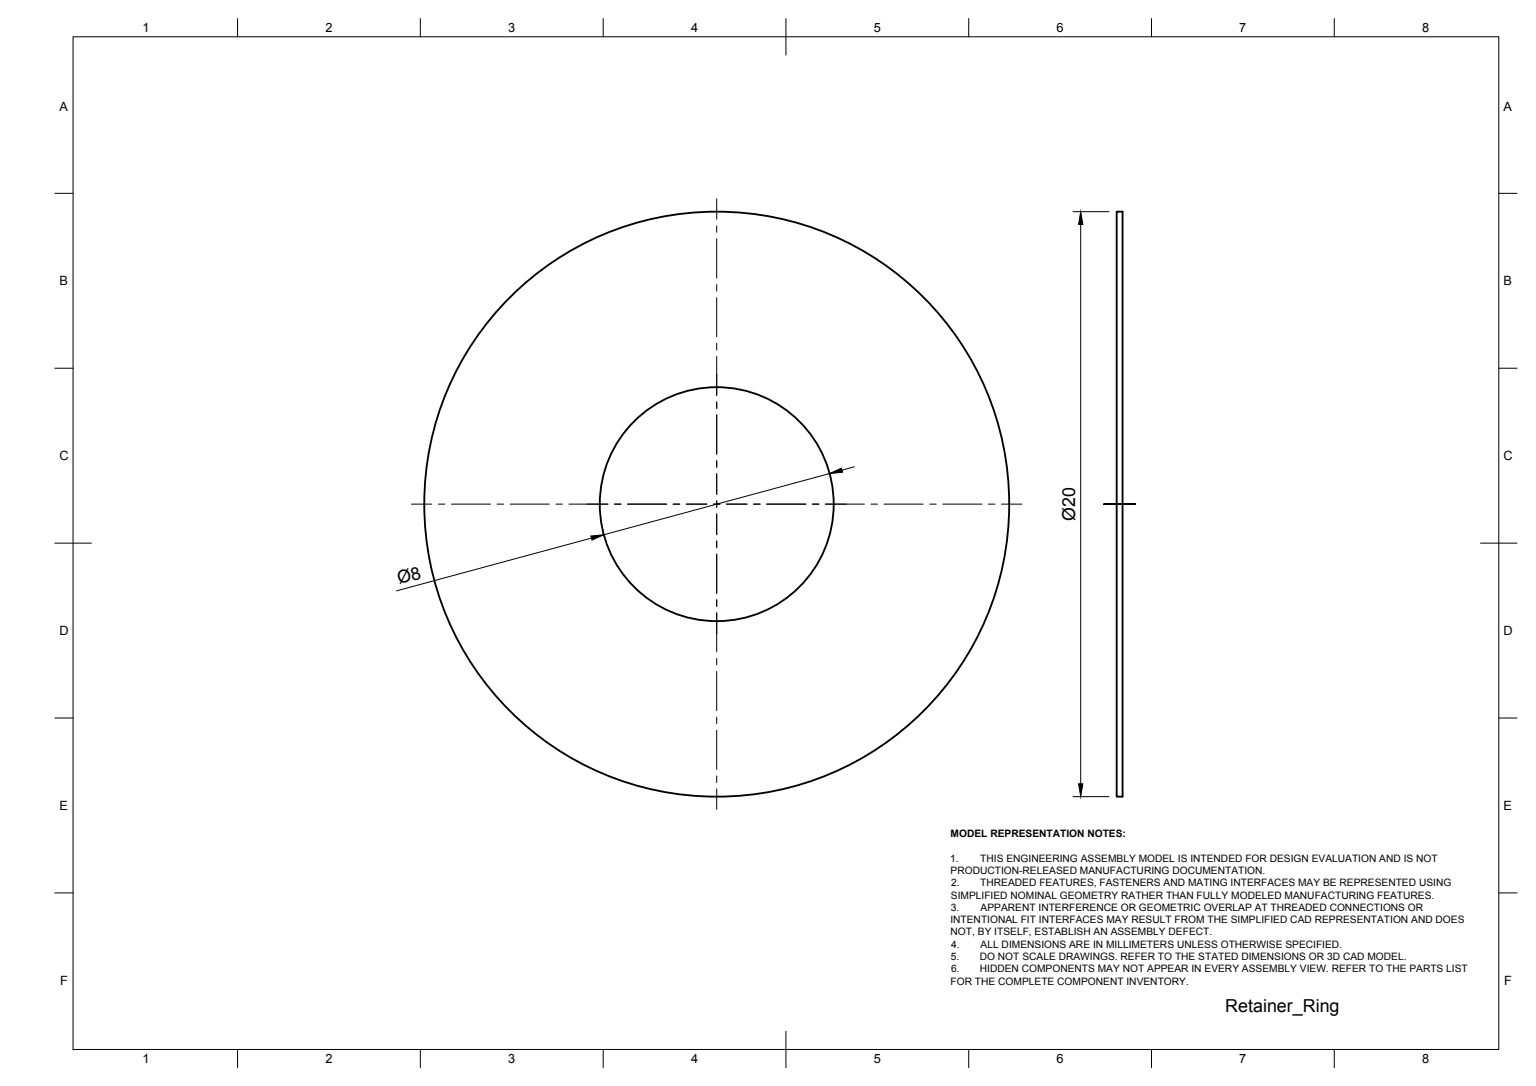
ISO-10303-21;
HEADER;
/* Generated by software containing ST-Developer
 * from STEP Tools, Inc. (www.steptools.com) 
 */

FILE_DESCRIPTION(
/* description */ (''),
/* implementation_level */ '2;1');

FILE_NAME(
/* name */ 'Retainer_Ring.step',
/* time_stamp */ '2026-10-06T12:52:28-07:00',
/* author */ (''),
/* organization */ (''),
/* preprocessor_version */ 'ST-DEVELOPER v20.2',
/* originating_system */ 'Autodesk Translation Framework v15.15.0.0',
/* authorisation */ '');

FILE_SCHEMA (('AUTOMOTIVE_DESIGN { 1 0 10303 214 3 1 1 }'));
ENDSEC;

DATA;
#10=MECHANICAL_DESIGN_GEOMETRIC_PRESENTATION_REPRESENTATION('',(#75),#34403);
#59=SHAPE_REPRESENTATION_RELATIONSHIP('SRR','None',#34437,#67);
#67=ADVANCED_BREP_SHAPE_REPRESENTATION('',(#83),#34397);
#75=STYLED_ITEM('',(#34484),#83);
#83=MANIFOLD_SOLID_BREP('Body1',#4384);
#95=FACE_BOUND('',#769,.T.);
#96=FACE_BOUND('',#771,.T.);
#129=PLANE('',#4520);
#130=PLANE('',#4521);
#178=CIRCLE('',#4515,4.);
#179=CIRCLE('',#4516,4.);
#180=CIRCLE('',#4518,10.);
#181=CIRCLE('',#4519,10.);
#529=FACE_OUTER_BOUND('',#766,.T.);
#530=FACE_OUTER_BOUND('',#767,.T.);
#531=FACE_OUTER_BOUND('',#768,.T.);
#532=FACE_OUTER_BOUND('',#770,.T.);
#766=EDGE_LOOP('',(#2745,#2746,#2747,#2748));
#767=EDGE_LOOP('',(#2749,#2750,#2751,#2752));
#768=EDGE_LOOP('',(#2753));
#769=EDGE_LOOP('',(#2754));
#770=EDGE_LOOP('',(#2755));
#771=EDGE_LOOP('',(#2756));
#1019=LINE('',#6398,#1156);
#1020=LINE('',#6404,#1157);
#1156=VECTOR('',#5082,4.);
#1157=VECTOR('',#5089,10.);
#1562=VERTEX_POINT('',#6395);
#1563=VERTEX_POINT('',#6397);
#1564=VERTEX_POINT('',#6401);
#1565=VERTEX_POINT('',#6403);
#2037=EDGE_CURVE('',#1562,#1562,#178,.T.);
#2038=EDGE_CURVE('',#1562,#1563,#1019,.T.);
#2039=EDGE_CURVE('',#1563,#1563,#179,.T.);
#2040=EDGE_CURVE('',#1564,#1564,#180,.F.);
#2041=EDGE_CURVE('',#1564,#1565,#1020,.T.);
#2042=EDGE_CURVE('',#1565,#1565,#181,.F.);
#2745=ORIENTED_EDGE('',*,*,#2037,.T.);
#2746=ORIENTED_EDGE('',*,*,#2038,.T.);
#2747=ORIENTED_EDGE('',*,*,#2039,.F.);
#2748=ORIENTED_EDGE('',*,*,#2038,.F.);
#2749=ORIENTED_EDGE('',*,*,#2040,.F.);
#2750=ORIENTED_EDGE('',*,*,#2041,.T.);
#2751=ORIENTED_EDGE('',*,*,#2042,.T.);
#2752=ORIENTED_EDGE('',*,*,#2041,.F.);
#2753=ORIENTED_EDGE('',*,*,#2040,.T.);
#2754=ORIENTED_EDGE('',*,*,#2039,.T.);
#2755=ORIENTED_EDGE('',*,*,#2042,.F.);
#2756=ORIENTED_EDGE('',*,*,#2037,.F.);
#4042=CYLINDRICAL_SURFACE('',#4514,4.);
#4043=CYLINDRICAL_SURFACE('',#4517,10.);
#4164=ADVANCED_FACE('',(#529),#4042,.F.);
#4165=ADVANCED_FACE('',(#530),#4043,.T.);
#4166=ADVANCED_FACE('',(#531,#95),#129,.T.);
#4167=ADVANCED_FACE('',(#532,#96),#130,.F.);
#4384=CLOSED_SHELL('',(#4164,#4165,#4166,#4167));
#4513=AXIS2_PLACEMENT_3D('',#6393,#5076,#5077);
#4514=AXIS2_PLACEMENT_3D('',#6394,#5078,#5079);
#4515=AXIS2_PLACEMENT_3D('',#6396,#5080,#5081);
#4516=AXIS2_PLACEMENT_3D('',#6399,#5083,#5084);
#4517=AXIS2_PLACEMENT_3D('',#6400,#5085,#5086);
#4518=AXIS2_PLACEMENT_3D('',#6402,#5087,#5088);
#4519=AXIS2_PLACEMENT_3D('',#6405,#5090,#5091);
#4520=AXIS2_PLACEMENT_3D('',#6406,#5092,#5093);
#4521=AXIS2_PLACEMENT_3D('',#6407,#5094,#5095);
#5076=DIRECTION('axis',(0.,0.,1.));
#5077=DIRECTION('refdir',(1.,0.,0.));
#5078=DIRECTION('center_axis',(0.,0.,1.));
#5079=DIRECTION('ref_axis',(-1.,0.,0.));
#5080=DIRECTION('center_axis',(0.,0.,-1.));
#5081=DIRECTION('ref_axis',(-1.,0.,0.));
#5082=DIRECTION('',(0.,0.,1.));
#5083=DIRECTION('center_axis',(0.,0.,-1.));
#5084=DIRECTION('ref_axis',(-1.,0.,0.));
#5085=DIRECTION('center_axis',(0.,0.,1.));
#5086=DIRECTION('ref_axis',(-1.,0.,0.));
#5087=DIRECTION('center_axis',(0.,0.,-1.));
#5088=DIRECTION('ref_axis',(-1.,0.,0.));
#5089=DIRECTION('',(0.,0.,-1.));
#5090=DIRECTION('center_axis',(0.,0.,-1.));
#5091=DIRECTION('ref_axis',(-1.,0.,0.));
#5092=DIRECTION('center_axis',(0.,0.,1.));
#5093=DIRECTION('ref_axis',(-1.,0.,0.));
#5094=DIRECTION('center_axis',(0.,0.,1.));
#5095=DIRECTION('ref_axis',(-1.,0.,0.));
#6393=CARTESIAN_POINT('',(0.,0.,0.));
#6394=CARTESIAN_POINT('Origin',(0.,0.,60.));
#6395=CARTESIAN_POINT('',(4.,4.89858719658941E-16,60.));
#6396=CARTESIAN_POINT('Origin',(0.,0.,60.));
#6397=CARTESIAN_POINT('',(4.,4.89858719658941E-16,60.2));
#6398=CARTESIAN_POINT('',(4.,4.89858719658941E-16,60.));
#6399=CARTESIAN_POINT('Origin',(0.,0.,60.2));
#6400=CARTESIAN_POINT('Origin',(0.,0.,60.));
#6401=CARTESIAN_POINT('',(10.,-1.22464679914735E-15,60.2));
#6402=CARTESIAN_POINT('Origin',(0.,0.,60.2));
#6403=CARTESIAN_POINT('',(10.,-1.22464679914735E-15,60.));
#6404=CARTESIAN_POINT('',(10.,1.22464679914735E-15,60.));
#6405=CARTESIAN_POINT('Origin',(0.,0.,60.));
#6406=CARTESIAN_POINT('Origin',(0.,0.,60.2));
#6407=CARTESIAN_POINT('Origin',(0.,0.,60.));
#34387=UNCERTAINTY_MEASURE_WITH_UNIT(LENGTH_MEASURE(0.01),#34404,
'DISTANCE_ACCURACY_VALUE',
'Maximum model space distance between geometric entities at asserted c
onnectivities');
#34393=UNCERTAINTY_MEASURE_WITH_UNIT(LENGTH_MEASURE(0.01),#34404,
'DISTANCE_ACCURACY_VALUE',
'Maximum model space distance between geometric entities at asserted c
onnectivities');
#34397=(
GEOMETRIC_REPRESENTATION_CONTEXT(3)
GLOBAL_UNCERTAINTY_ASSIGNED_CONTEXT((#34387))
GLOBAL_UNIT_ASSIGNED_CONTEXT((#34404,#34406,#34407))
REPRESENTATION_CONTEXT('','3D')
);
#34403=(
GEOMETRIC_REPRESENTATION_CONTEXT(3)
GLOBAL_UNCERTAINTY_ASSIGNED_CONTEXT((#34393))
GLOBAL_UNIT_ASSIGNED_CONTEXT((#34404,#34406,#34407))
REPRESENTATION_CONTEXT('','3D')
);
#34404=(
LENGTH_UNIT()
NAMED_UNIT(*)
SI_UNIT(.MILLI.,.METRE.)
);
#34406=(
NAMED_UNIT(*)
PLANE_ANGLE_UNIT()
SI_UNIT($,.RADIAN.)
);
#34407=(
NAMED_UNIT(*)
SI_UNIT($,.STERADIAN.)
SOLID_ANGLE_UNIT()
);
#34411=SHAPE_DEFINITION_REPRESENTATION(#34420,#34437);
#34420=PRODUCT_DEFINITION_SHAPE('',$,#34447);
#34437=SHAPE_REPRESENTATION('',(#4513),#34397);
#34443=PRODUCT_DEFINITION_CONTEXT('part definition',#34472,'design');
#34447=PRODUCT_DEFINITION('Retainer_Ring','Retainer_Ring',#34456,#34443);
#34456=PRODUCT_DEFINITION_FORMATION('',$,#34477);
#34472=APPLICATION_CONTEXT(
'Core Data for Automotive Mechanical Design Process');
#34473=PRODUCT_CONTEXT('part definition',#34472,'mechanical');
#34477=PRODUCT('Retainer_Ring','Retainer_Ring',$,(#34473));
#34484=PRESENTATION_STYLE_ASSIGNMENT((#34486));
#34486=SURFACE_STYLE_USAGE(.BOTH.,#34488);
#34488=SURFACE_SIDE_STYLE('',(#34490));
#34490=SURFACE_STYLE_FILL_AREA(#34492);
#34492=FILL_AREA_STYLE('Opaque(160,160,160)',(#34494));
#34494=FILL_AREA_STYLE_COLOUR('Opaque(160,160,160)',#34496);
#34496=COLOUR_RGB('Opaque(160,160,160)', 0.09019608, 0.27058824, 0.51372549);
ENDSEC;
END-ISO-10303-21;
